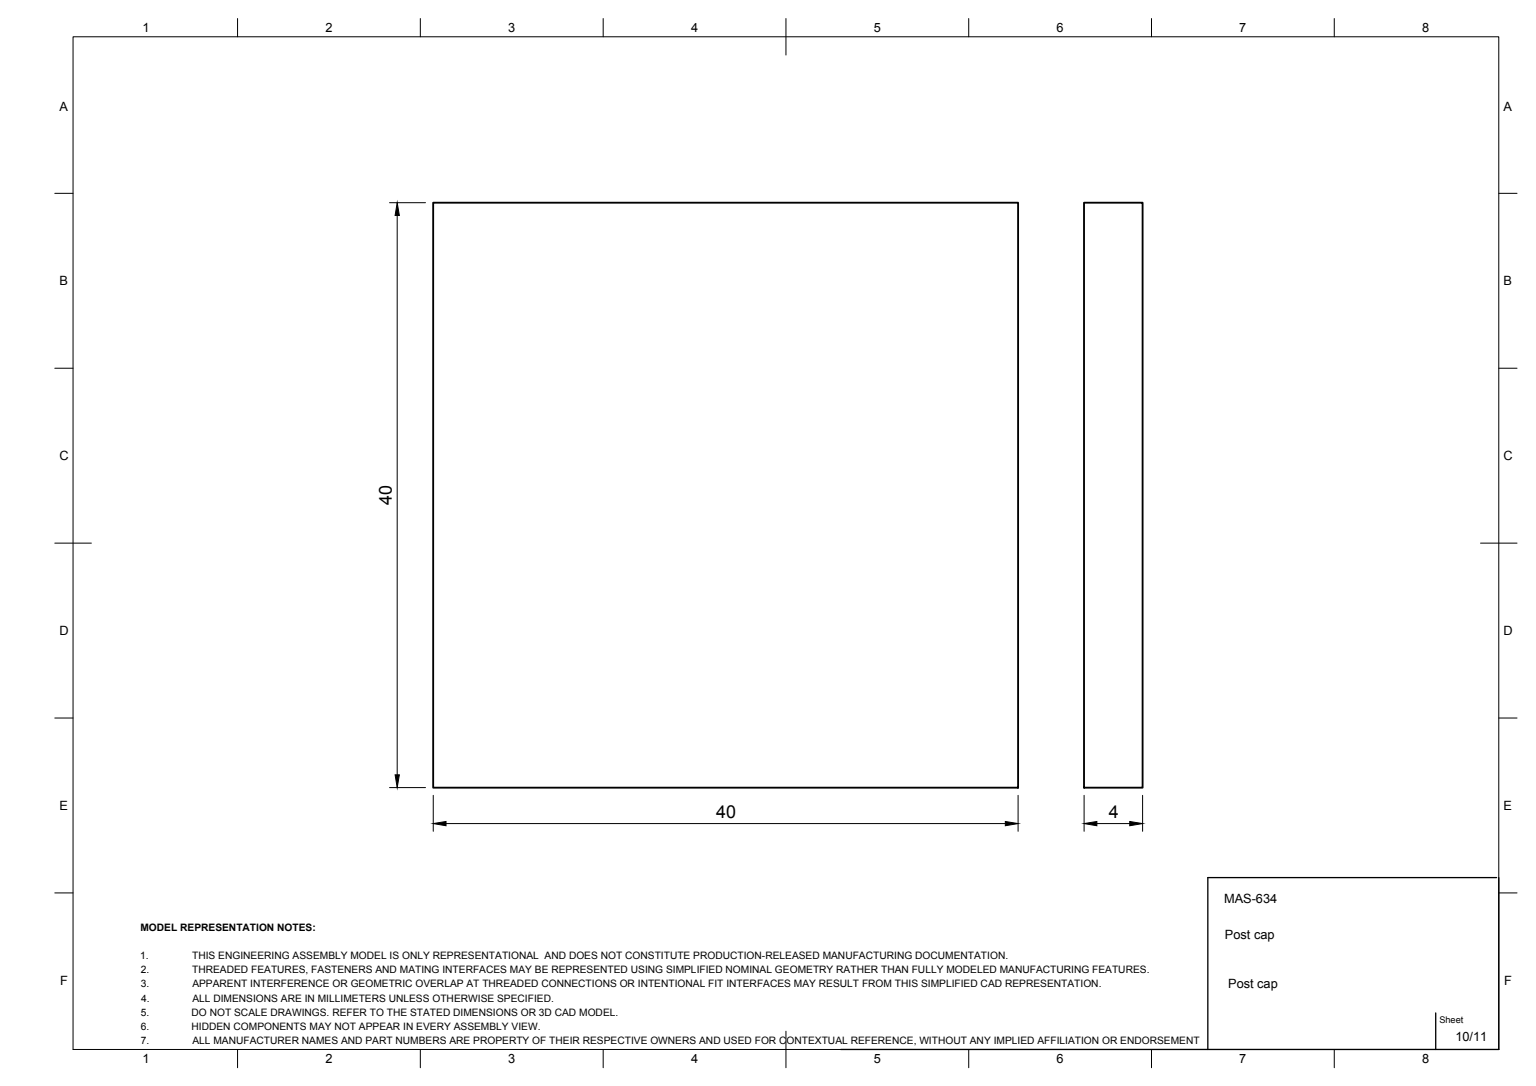
ISO-10303-21;
HEADER;
/* Generated by software containing ST-Developer
 * from STEP Tools, Inc. (www.steptools.com) 
 */

FILE_DESCRIPTION(
/* description */ ('Independent AHU equipment rack. Nominal800x600 frame on1000long40squa
re aluminum posts; two removable notched shelves; welded perimeter/cro
ss rails and rear gussets; two mounting channels; four isolation pads 
and anchor-ready feet. Imported native extrusion library retained and 
cut-length parameters customized per family. Shelf hardware uses model
ed M6 rivet nuts and screws. Weld design, floor anchors and load ratin
g require engineering selection.'),
/* implementation_level */ '2;1');

FILE_NAME(
/* name */ 'Post cap.step',
/* time_stamp */ '2026-11-07T19:04:45-08:00',
/* author */ (''),
/* organization */ (''),
/* preprocessor_version */ 'ST-DEVELOPER v20.2',
/* originating_system */ 'Autodesk Translation Framework v15.17.0.0',
/* authorisation */ '');

FILE_SCHEMA (('AUTOMOTIVE_DESIGN { 1 0 10303 214 3 1 1 }'));
ENDSEC;

DATA;
#10=MECHANICAL_DESIGN_GEOMETRIC_PRESENTATION_REPRESENTATION('',(#342),#9777);
#320=SHAPE_REPRESENTATION_RELATIONSHIP('SRR','None',#9864,#331);
#331=ADVANCED_BREP_SHAPE_REPRESENTATION('',(#353),#9773);
#342=STYLED_ITEM('',(#9927),#353);
#353=MANIFOLD_SOLID_BREP('Body1',#3847);
#476=PLANE('',#4204);
#477=PLANE('',#4205);
#478=PLANE('',#4206);
#479=PLANE('',#4207);
#480=PLANE('',#4208);
#481=PLANE('',#4209);
#620=FACE_OUTER_BOUND('',#864,.T.);
#621=FACE_OUTER_BOUND('',#865,.T.);
#622=FACE_OUTER_BOUND('',#866,.T.);
#623=FACE_OUTER_BOUND('',#867,.T.);
#624=FACE_OUTER_BOUND('',#868,.T.);
#625=FACE_OUTER_BOUND('',#869,.T.);
#864=EDGE_LOOP('',(#3139,#3140,#3141,#3142));
#865=EDGE_LOOP('',(#3143,#3144,#3145,#3146));
#866=EDGE_LOOP('',(#3147,#3148,#3149,#3150));
#867=EDGE_LOOP('',(#3151,#3152,#3153,#3154));
#868=EDGE_LOOP('',(#3155,#3156,#3157,#3158));
#869=EDGE_LOOP('',(#3159,#3160,#3161,#3162));
#1159=LINE('',#6053,#1452);
#1160=LINE('',#6055,#1453);
#1161=LINE('',#6057,#1454);
#1162=LINE('',#6058,#1455);
#1163=LINE('',#6061,#1456);
#1164=LINE('',#6063,#1457);
#1165=LINE('',#6064,#1458);
#1166=LINE('',#6067,#1459);
#1167=LINE('',#6069,#1460);
#1168=LINE('',#6070,#1461);
#1169=LINE('',#6072,#1462);
#1170=LINE('',#6073,#1463);
#1452=VECTOR('',#5024,10.);
#1453=VECTOR('',#5025,10.);
#1454=VECTOR('',#5026,10.);
#1455=VECTOR('',#5027,10.);
#1456=VECTOR('',#5030,10.);
#1457=VECTOR('',#5031,10.);
#1458=VECTOR('',#5032,10.);
#1459=VECTOR('',#5035,10.);
#1460=VECTOR('',#5036,10.);
#1461=VECTOR('',#5037,10.);
#1462=VECTOR('',#5040,10.);
#1463=VECTOR('',#5041,10.);
#1868=VERTEX_POINT('',#6051);
#1869=VERTEX_POINT('',#6052);
#1870=VERTEX_POINT('',#6054);
#1871=VERTEX_POINT('',#6056);
#1872=VERTEX_POINT('',#6060);
#1873=VERTEX_POINT('',#6062);
#1874=VERTEX_POINT('',#6066);
#1875=VERTEX_POINT('',#6068);
#2314=EDGE_CURVE('',#1868,#1869,#1159,.T.);
#2315=EDGE_CURVE('',#1869,#1870,#1160,.T.);
#2316=EDGE_CURVE('',#1871,#1870,#1161,.T.);
#2317=EDGE_CURVE('',#1868,#1871,#1162,.T.);
#2318=EDGE_CURVE('',#1872,#1868,#1163,.T.);
#2319=EDGE_CURVE('',#1873,#1871,#1164,.T.);
#2320=EDGE_CURVE('',#1872,#1873,#1165,.T.);
#2321=EDGE_CURVE('',#1874,#1872,#1166,.T.);
#2322=EDGE_CURVE('',#1875,#1873,#1167,.T.);
#2323=EDGE_CURVE('',#1874,#1875,#1168,.T.);
#2324=EDGE_CURVE('',#1869,#1874,#1169,.T.);
#2325=EDGE_CURVE('',#1870,#1875,#1170,.T.);
#3139=ORIENTED_EDGE('',*,*,#2314,.T.);
#3140=ORIENTED_EDGE('',*,*,#2315,.T.);
#3141=ORIENTED_EDGE('',*,*,#2316,.F.);
#3142=ORIENTED_EDGE('',*,*,#2317,.F.);
#3143=ORIENTED_EDGE('',*,*,#2318,.T.);
#3144=ORIENTED_EDGE('',*,*,#2317,.T.);
#3145=ORIENTED_EDGE('',*,*,#2319,.F.);
#3146=ORIENTED_EDGE('',*,*,#2320,.F.);
#3147=ORIENTED_EDGE('',*,*,#2321,.T.);
#3148=ORIENTED_EDGE('',*,*,#2320,.T.);
#3149=ORIENTED_EDGE('',*,*,#2322,.F.);
#3150=ORIENTED_EDGE('',*,*,#2323,.F.);
#3151=ORIENTED_EDGE('',*,*,#2324,.T.);
#3152=ORIENTED_EDGE('',*,*,#2323,.T.);
#3153=ORIENTED_EDGE('',*,*,#2325,.F.);
#3154=ORIENTED_EDGE('',*,*,#2315,.F.);
#3155=ORIENTED_EDGE('',*,*,#2325,.T.);
#3156=ORIENTED_EDGE('',*,*,#2322,.T.);
#3157=ORIENTED_EDGE('',*,*,#2319,.T.);
#3158=ORIENTED_EDGE('',*,*,#2316,.T.);
#3159=ORIENTED_EDGE('',*,*,#2324,.F.);
#3160=ORIENTED_EDGE('',*,*,#2314,.F.);
#3161=ORIENTED_EDGE('',*,*,#2318,.F.);
#3162=ORIENTED_EDGE('',*,*,#2321,.F.);
#3760=ADVANCED_FACE('',(#620),#476,.T.);
#3761=ADVANCED_FACE('',(#621),#477,.T.);
#3762=ADVANCED_FACE('',(#622),#478,.T.);
#3763=ADVANCED_FACE('',(#623),#479,.T.);
#3764=ADVANCED_FACE('',(#624),#480,.T.);
#3765=ADVANCED_FACE('',(#625),#481,.F.);
#3847=CLOSED_SHELL('',(#3760,#3761,#3762,#3763,#3764,#3765));
#4203=AXIS2_PLACEMENT_3D('',#6049,#5020,#5021);
#4204=AXIS2_PLACEMENT_3D('',#6050,#5022,#5023);
#4205=AXIS2_PLACEMENT_3D('',#6059,#5028,#5029);
#4206=AXIS2_PLACEMENT_3D('',#6065,#5033,#5034);
#4207=AXIS2_PLACEMENT_3D('',#6071,#5038,#5039);
#4208=AXIS2_PLACEMENT_3D('',#6074,#5042,#5043);
#4209=AXIS2_PLACEMENT_3D('',#6075,#5044,#5045);
#5020=DIRECTION('axis',(0.,0.,1.));
#5021=DIRECTION('refdir',(1.,0.,0.));
#5022=DIRECTION('center_axis',(0.,1.,0.));
#5023=DIRECTION('ref_axis',(-1.,0.,0.));
#5024=DIRECTION('',(-1.,0.,0.));
#5025=DIRECTION('',(0.,0.,1.));
#5026=DIRECTION('',(-1.,0.,0.));
#5027=DIRECTION('',(0.,0.,1.));
#5028=DIRECTION('center_axis',(1.,0.,0.));
#5029=DIRECTION('ref_axis',(0.,1.,0.));
#5030=DIRECTION('',(0.,1.,0.));
#5031=DIRECTION('',(0.,1.,0.));
#5032=DIRECTION('',(0.,0.,1.));
#5033=DIRECTION('center_axis',(0.,-1.,0.));
#5034=DIRECTION('ref_axis',(1.,0.,0.));
#5035=DIRECTION('',(1.,0.,0.));
#5036=DIRECTION('',(1.,0.,0.));
#5037=DIRECTION('',(0.,0.,1.));
#5038=DIRECTION('center_axis',(-1.,0.,0.));
#5039=DIRECTION('ref_axis',(0.,-1.,0.));
#5040=DIRECTION('',(0.,-1.,0.));
#5041=DIRECTION('',(0.,-1.,0.));
#5042=DIRECTION('center_axis',(0.,0.,1.));
#5043=DIRECTION('ref_axis',(1.,0.,0.));
#5044=DIRECTION('center_axis',(0.,0.,1.));
#5045=DIRECTION('ref_axis',(1.,0.,0.));
#6049=CARTESIAN_POINT('',(0.,0.,0.));
#6050=CARTESIAN_POINT('Origin',(20.,20.,0.));
#6051=CARTESIAN_POINT('',(20.,20.,0.));
#6052=CARTESIAN_POINT('',(-20.,20.,0.));
#6053=CARTESIAN_POINT('',(20.,20.,0.));
#6054=CARTESIAN_POINT('',(-20.,20.,4.));
#6055=CARTESIAN_POINT('',(-20.,20.,0.));
#6056=CARTESIAN_POINT('',(20.,20.,4.));
#6057=CARTESIAN_POINT('',(20.,20.,4.));
#6058=CARTESIAN_POINT('',(20.,20.,0.));
#6059=CARTESIAN_POINT('Origin',(20.,-20.,0.));
#6060=CARTESIAN_POINT('',(20.,-20.,0.));
#6061=CARTESIAN_POINT('',(20.,-20.,0.));
#6062=CARTESIAN_POINT('',(20.,-20.,4.));
#6063=CARTESIAN_POINT('',(20.,-20.,4.));
#6064=CARTESIAN_POINT('',(20.,-20.,0.));
#6065=CARTESIAN_POINT('Origin',(-20.,-20.,0.));
#6066=CARTESIAN_POINT('',(-20.,-20.,0.));
#6067=CARTESIAN_POINT('',(-20.,-20.,0.));
#6068=CARTESIAN_POINT('',(-20.,-20.,4.));
#6069=CARTESIAN_POINT('',(-20.,-20.,4.));
#6070=CARTESIAN_POINT('',(-20.,-20.,0.));
#6071=CARTESIAN_POINT('Origin',(-20.,20.,0.));
#6072=CARTESIAN_POINT('',(-20.,20.,0.));
#6073=CARTESIAN_POINT('',(-20.,20.,4.));
#6074=CARTESIAN_POINT('Origin',(0.,0.,4.));
#6075=CARTESIAN_POINT('Origin',(0.,0.,0.));
#9760=UNCERTAINTY_MEASURE_WITH_UNIT(LENGTH_MEASURE(0.01),#9778,
'DISTANCE_ACCURACY_VALUE',
'Maximum model space distance between geometric entities at asserted c
onnectivities');
#9764=UNCERTAINTY_MEASURE_WITH_UNIT(LENGTH_MEASURE(0.01),#9778,
'DISTANCE_ACCURACY_VALUE',
'Maximum model space distance between geometric entities at asserted c
onnectivities');
#9773=(
GEOMETRIC_REPRESENTATION_CONTEXT(3)
GLOBAL_UNCERTAINTY_ASSIGNED_CONTEXT((#9760))
GLOBAL_UNIT_ASSIGNED_CONTEXT((#9778,#9780,#9781))
REPRESENTATION_CONTEXT('','3D')
);
#9777=(
GEOMETRIC_REPRESENTATION_CONTEXT(3)
GLOBAL_UNCERTAINTY_ASSIGNED_CONTEXT((#9764))
GLOBAL_UNIT_ASSIGNED_CONTEXT((#9778,#9780,#9781))
REPRESENTATION_CONTEXT('','3D')
);
#9778=(
LENGTH_UNIT()
NAMED_UNIT(*)
SI_UNIT(.MILLI.,.METRE.)
);
#9780=(
NAMED_UNIT(*)
PLANE_ANGLE_UNIT()
SI_UNIT($,.RADIAN.)
);
#9781=(
NAMED_UNIT(*)
SI_UNIT($,.STERADIAN.)
SOLID_ANGLE_UNIT()
);
#9790=SHAPE_DEFINITION_REPRESENTATION(#9802,#9864);
#9802=PRODUCT_DEFINITION_SHAPE('',$,#9877);
#9864=SHAPE_REPRESENTATION('',(#4203),#9773);
#9868=PRODUCT_DEFINITION_CONTEXT('part definition',#9906,'design');
#9877=PRODUCT_DEFINITION('Post cap','Post cap',#9889,#9868);
#9889=PRODUCT_DEFINITION_FORMATION('',$,#9916);
#9906=APPLICATION_CONTEXT(
'Core Data for Automotive Mechanical Design Process');
#9907=PRODUCT_CONTEXT('part definition',#9906,'mechanical');
#9916=PRODUCT('Post cap','Post cap',$,(#9907));
#9927=PRESENTATION_STYLE_ASSIGNMENT((#9938));
#9938=SURFACE_STYLE_USAGE(.BOTH.,#9949);
#9949=SURFACE_SIDE_STYLE('',(#9960));
#9960=SURFACE_STYLE_FILL_AREA(#9971);
#9971=FILL_AREA_STYLE('Cap gray',(#9982));
#9982=FILL_AREA_STYLE_COLOUR('Cap gray',#9993);
#9993=COLOUR_RGB('Cap gray',0.725490196078431,0.752941176470588,0.792156862745098);
ENDSEC;
END-ISO-10303-21;
